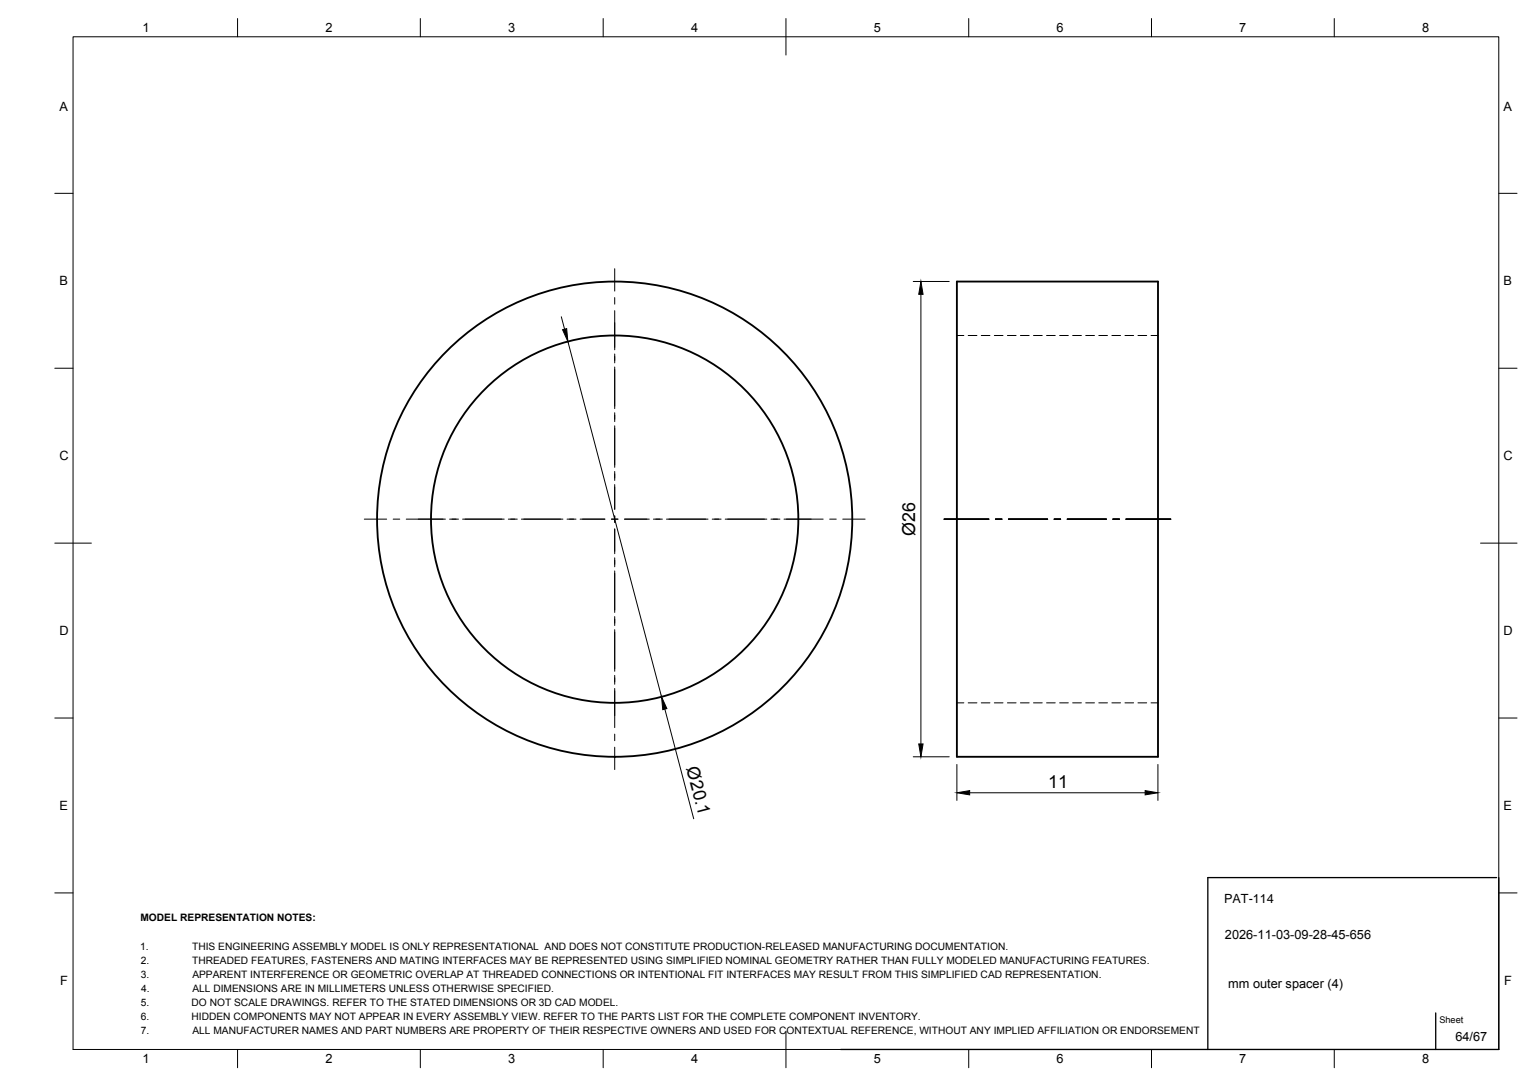
ISO-10303-21;
HEADER;
/* Generated by software containing ST-Developer
 * from STEP Tools, Inc. (www.steptools.com) 
 */

FILE_DESCRIPTION(
/* description */ ('Two-stage gear reducer in split housing'),
/* implementation_level */ '2;1');

FILE_NAME(
/* name */ 'mm outer spacer (4).step',
/* time_stamp */ '2026-10-28T03:22:31-07:00',
/* author */ (''),
/* organization */ (''),
/* preprocessor_version */ 'ST-DEVELOPER v20.2',
/* originating_system */ 'Autodesk Translation Framework v15.17.0.0',
/* authorisation */ '');

FILE_SCHEMA (('AUTOMOTIVE_DESIGN { 1 0 10303 214 3 1 1 }'));
ENDSEC;

DATA;
#10=MECHANICAL_DESIGN_GEOMETRIC_PRESENTATION_REPRESENTATION('',(#1298),#73366);
#1171=SHAPE_REPRESENTATION_RELATIONSHIP('SRR','None',#73663,#1227);
#1227=ADVANCED_BREP_SHAPE_REPRESENTATION('',(#1367),#73359);
#1298=STYLED_ITEM('',(#73974),#1367);
#1367=MANIFOLD_SOLID_BREP('Body1',#16188);
#1590=FACE_BOUND('',#3841,.T.);
#1591=FACE_BOUND('',#3843,.T.);
#1929=PLANE('',#18188);
#1930=PLANE('',#18189);
#2709=FACE_OUTER_BOUND('',#3838,.T.);
#2710=FACE_OUTER_BOUND('',#3839,.T.);
#2711=FACE_OUTER_BOUND('',#3840,.T.);
#2712=FACE_OUTER_BOUND('',#3842,.T.);
#3838=EDGE_LOOP('',(#13771,#13772,#13773,#13774));
#3839=EDGE_LOOP('',(#13775,#13776,#13777,#13778));
#3840=EDGE_LOOP('',(#13779));
#3841=EDGE_LOOP('',(#13780));
#3842=EDGE_LOOP('',(#13781));
#3843=EDGE_LOOP('',(#13782));
#4856=LINE('',#49485,#5880);
#4857=LINE('',#49491,#5881);
#5880=VECTOR('',#22002,1.005);
#5881=VECTOR('',#22009,1.3);
#6720=CIRCLE('',#18183,1.005);
#6721=CIRCLE('',#18184,1.005);
#6722=CIRCLE('',#18186,1.3);
#6723=CIRCLE('',#18187,1.3);
#7929=VERTEX_POINT('',#49482);
#7930=VERTEX_POINT('',#49484);
#7931=VERTEX_POINT('',#49488);
#7932=VERTEX_POINT('',#49490);
#9939=EDGE_CURVE('',#7929,#7929,#6720,.T.);
#9940=EDGE_CURVE('',#7929,#7930,#4856,.T.);
#9941=EDGE_CURVE('',#7930,#7930,#6721,.T.);
#9942=EDGE_CURVE('',#7931,#7931,#6722,.T.);
#9943=EDGE_CURVE('',#7931,#7932,#4857,.T.);
#9944=EDGE_CURVE('',#7932,#7932,#6723,.T.);
#13771=ORIENTED_EDGE('',*,*,#9939,.F.);
#13772=ORIENTED_EDGE('',*,*,#9940,.T.);
#13773=ORIENTED_EDGE('',*,*,#9941,.T.);
#13774=ORIENTED_EDGE('',*,*,#9940,.F.);
#13775=ORIENTED_EDGE('',*,*,#9942,.F.);
#13776=ORIENTED_EDGE('',*,*,#9943,.T.);
#13777=ORIENTED_EDGE('',*,*,#9944,.T.);
#13778=ORIENTED_EDGE('',*,*,#9943,.F.);
#13779=ORIENTED_EDGE('',*,*,#9942,.T.);
#13780=ORIENTED_EDGE('',*,*,#9939,.T.);
#13781=ORIENTED_EDGE('',*,*,#9944,.F.);
#13782=ORIENTED_EDGE('',*,*,#9941,.F.);
#15158=CYLINDRICAL_SURFACE('',#18182,1.005);
#15159=CYLINDRICAL_SURFACE('',#18185,1.3);
#15916=ADVANCED_FACE('',(#2709),#15158,.F.);
#15917=ADVANCED_FACE('',(#2710),#15159,.T.);
#15918=ADVANCED_FACE('',(#2711,#1590),#1929,.T.);
#15919=ADVANCED_FACE('',(#2712,#1591),#1930,.F.);
#16188=CLOSED_SHELL('',(#15916,#15917,#15918,#15919));
#18181=AXIS2_PLACEMENT_3D('',#49480,#21996,#21997);
#18182=AXIS2_PLACEMENT_3D('',#49481,#21998,#21999);
#18183=AXIS2_PLACEMENT_3D('',#49483,#22000,#22001);
#18184=AXIS2_PLACEMENT_3D('',#49486,#22003,#22004);
#18185=AXIS2_PLACEMENT_3D('',#49487,#22005,#22006);
#18186=AXIS2_PLACEMENT_3D('',#49489,#22007,#22008);
#18187=AXIS2_PLACEMENT_3D('',#49492,#22010,#22011);
#18188=AXIS2_PLACEMENT_3D('',#49493,#22012,#22013);
#18189=AXIS2_PLACEMENT_3D('',#49494,#22014,#22015);
#21996=DIRECTION('axis',(0.,0.,1.));
#21997=DIRECTION('refdir',(1.,0.,0.));
#21998=DIRECTION('center_axis',(0.,1.,0.));
#21999=DIRECTION('ref_axis',(1.,0.,0.));
#22000=DIRECTION('center_axis',(0.,-1.,0.));
#22001=DIRECTION('ref_axis',(1.,0.,0.));
#22002=DIRECTION('',(0.,-1.,0.));
#22003=DIRECTION('center_axis',(0.,-1.,0.));
#22004=DIRECTION('ref_axis',(1.,0.,0.));
#22005=DIRECTION('center_axis',(0.,1.,0.));
#22006=DIRECTION('ref_axis',(1.,0.,0.));
#22007=DIRECTION('center_axis',(0.,1.,0.));
#22008=DIRECTION('ref_axis',(1.,0.,0.));
#22009=DIRECTION('',(0.,-1.,0.));
#22010=DIRECTION('center_axis',(0.,1.,0.));
#22011=DIRECTION('ref_axis',(1.,0.,0.));
#22012=DIRECTION('center_axis',(0.,1.,0.));
#22013=DIRECTION('ref_axis',(1.,0.,0.));
#22014=DIRECTION('center_axis',(0.,1.,0.));
#22015=DIRECTION('ref_axis',(1.,0.,0.));
#49480=CARTESIAN_POINT('',(0.,0.,0.));
#49481=CARTESIAN_POINT('Origin',(12.,-7.8,10.));
#49482=CARTESIAN_POINT('',(10.995,-6.7,10.));
#49483=CARTESIAN_POINT('Origin',(12.,-6.7,10.));
#49484=CARTESIAN_POINT('',(10.995,-7.8,10.));
#49485=CARTESIAN_POINT('',(10.995,-7.8,10.));
#49486=CARTESIAN_POINT('Origin',(12.,-7.8,10.));
#49487=CARTESIAN_POINT('Origin',(12.,-7.8,10.));
#49488=CARTESIAN_POINT('',(10.7,-6.7,10.));
#49489=CARTESIAN_POINT('Origin',(12.,-6.7,10.));
#49490=CARTESIAN_POINT('',(10.7,-7.8,10.));
#49491=CARTESIAN_POINT('',(10.7,-7.8,10.));
#49492=CARTESIAN_POINT('Origin',(12.,-7.8,10.));
#49493=CARTESIAN_POINT('Origin',(12.,-6.7,10.));
#49494=CARTESIAN_POINT('Origin',(12.,-7.8,10.));
#73295=UNCERTAINTY_MEASURE_WITH_UNIT(LENGTH_MEASURE(0.001),#73367,
'DISTANCE_ACCURACY_VALUE',
'Maximum model space distance between geometric entities at asserted c
onnectivities');
#73302=UNCERTAINTY_MEASURE_WITH_UNIT(LENGTH_MEASURE(0.001),#73367,
'DISTANCE_ACCURACY_VALUE',
'Maximum model space distance between geometric entities at asserted c
onnectivities');
#73359=(
GEOMETRIC_REPRESENTATION_CONTEXT(3)
GLOBAL_UNCERTAINTY_ASSIGNED_CONTEXT((#73295))
GLOBAL_UNIT_ASSIGNED_CONTEXT((#73367,#73369,#73370))
REPRESENTATION_CONTEXT('','3D')
);
#73366=(
GEOMETRIC_REPRESENTATION_CONTEXT(3)
GLOBAL_UNCERTAINTY_ASSIGNED_CONTEXT((#73302))
GLOBAL_UNIT_ASSIGNED_CONTEXT((#73367,#73369,#73370))
REPRESENTATION_CONTEXT('','3D')
);
#73367=(
LENGTH_UNIT()
NAMED_UNIT(*)
SI_UNIT(.CENTI.,.METRE.)
);
#73369=(
NAMED_UNIT(*)
PLANE_ANGLE_UNIT()
SI_UNIT($,.RADIAN.)
);
#73370=(
NAMED_UNIT(*)
SI_UNIT($,.STERADIAN.)
SOLID_ANGLE_UNIT()
);
#73427=SHAPE_DEFINITION_REPRESENTATION(#73560,#73663);
#73560=PRODUCT_DEFINITION_SHAPE('',$,#73727);
#73663=SHAPE_REPRESENTATION('',(#18181),#73359);
#73670=PRODUCT_DEFINITION_CONTEXT('part definition',#73861,'design');
#73727=PRODUCT_DEFINITION('mm outer spacer (4)','mm outer spacer (4)',#73790,
#73670);
#73790=PRODUCT_DEFINITION_FORMATION('',$,#73919);
#73861=APPLICATION_CONTEXT(
'Core Data for Automotive Mechanical Design Process');
#73862=PRODUCT_CONTEXT('part definition',#73861,'mechanical');
#73919=PRODUCT('mm outer spacer (4)','mm outer spacer (4)',
'mm outer spacer (4)',(#73862));
#73968=COLOUR_RGB('Light Blue',0.38,0.62,0.78);
#73969=FILL_AREA_STYLE_COLOUR('',#73968);
#73970=FILL_AREA_STYLE('',(#73969));
#73971=SURFACE_STYLE_FILL_AREA(#73970);
#73972=SURFACE_SIDE_STYLE('',(#73971));
#73973=SURFACE_STYLE_USAGE(.BOTH.,#73972);
#73974=PRESENTATION_STYLE_ASSIGNMENT((#73973));
ENDSEC;
END-ISO-10303-21;
